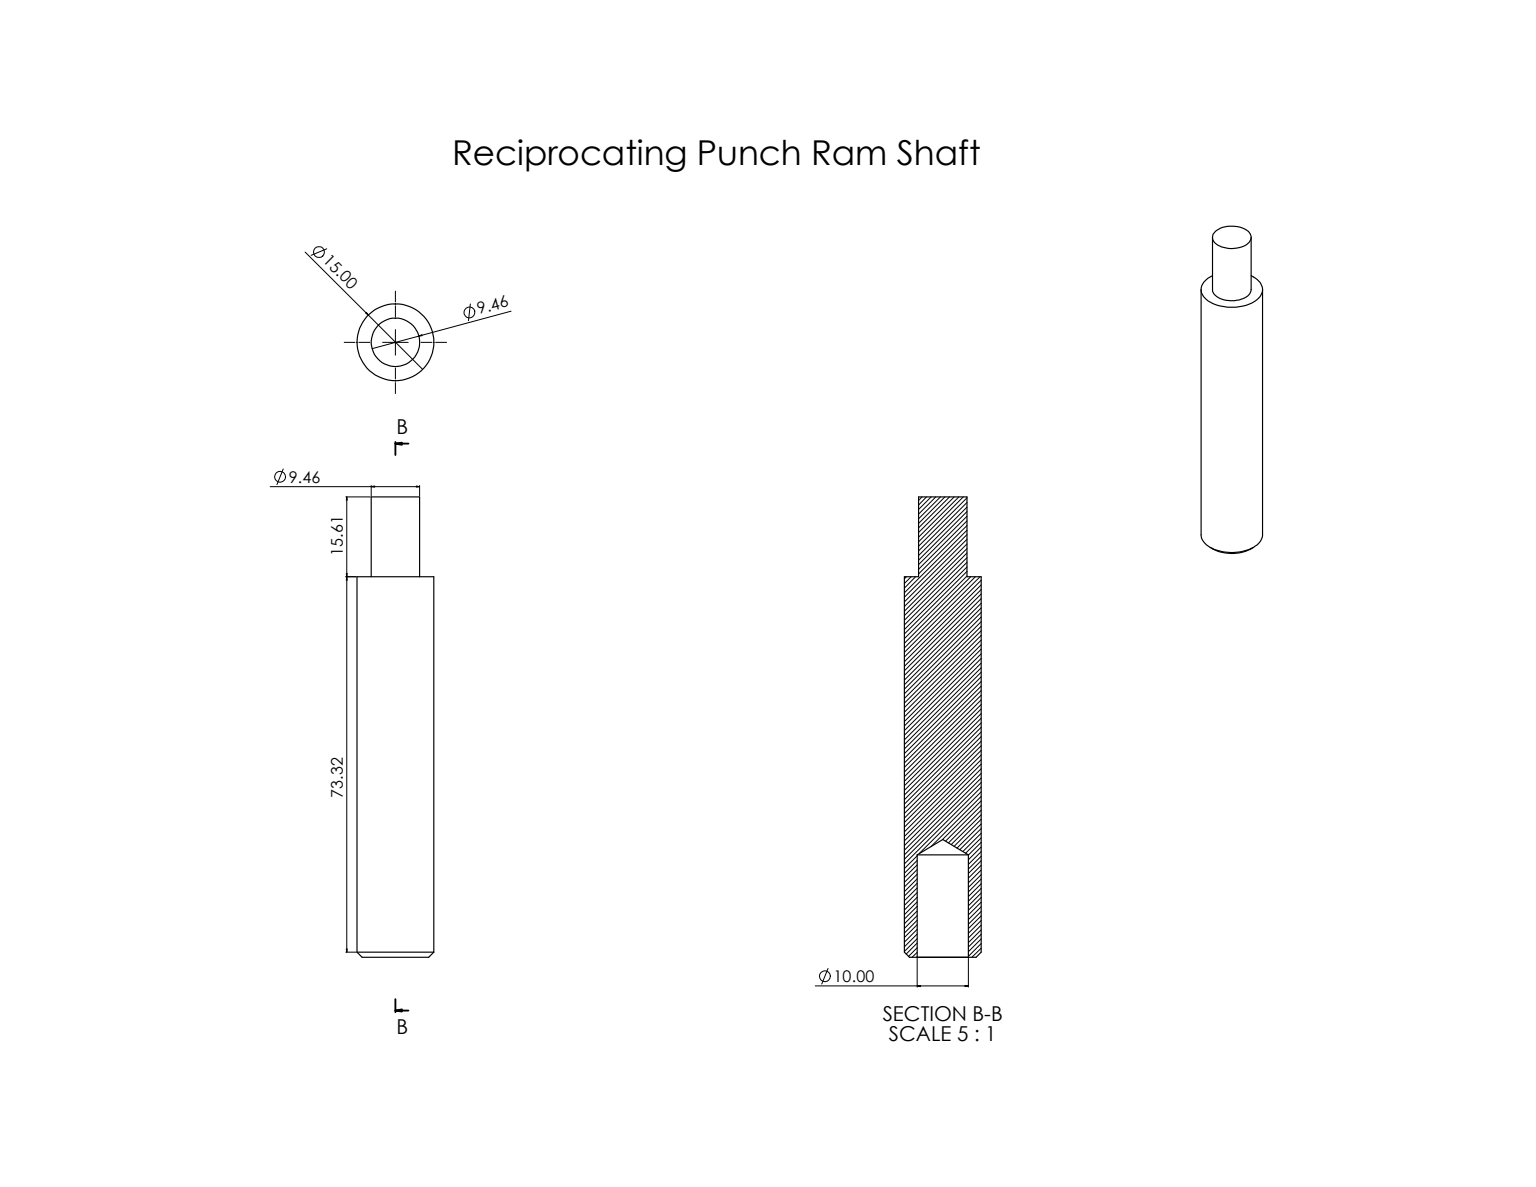
ISO-10303-21;
HEADER;
FILE_DESCRIPTION (('STEP AP214'),
    '1' );
FILE_NAME ('Reciprocating Punch Ram Shaft.step',
    '2026-10-20T14:49:59',
    ( '' ),
    ( '' ),
    'SwSTEP 2.0',
    'SolidWorks 2025',
    '' );
FILE_SCHEMA (( 'AUTOMOTIVE_DESIGN' ));
ENDSEC;

DATA;
#60=ORIENTED_EDGE ( 'NONE', *, *, #10146, .T. ) ;
#83=CIRCLE ( 'NONE', #590, 5.025000000000002132 ) ;
#136=CARTESIAN_POINT ( 'NONE',  ( -16.29350689640809691, -8.635287962196477096, 0.000000000000000000 ) ) ;
#199=DIRECTION ( 'NONE',  ( 0.000000000000000000, 0.000000000000000000, -1.000000000000000000 ) ) ;
#202=DIRECTION ( 'NONE',  ( 0.000000000000000000, 0.000000000000000000, -1.000000000000000000 ) ) ;
#307=CLOSED_SHELL ( 'NONE', ( #4177, #2796, #9152, #8006, #10397, #7112, #488, #9693, #5992, #7606, #7526, #5005, #9842, #7992, #7050 ) ) ;
#333=CARTESIAN_POINT ( 'NONE',  ( -16.29350689640809691, 81.26698356513965393, -4.729641367753003145 ) ) ;
#342=DIRECTION ( 'NONE',  ( 0.000000000000000000, 0.000000000000000000, -1.000000000000000000 ) ) ;
#358=DIRECTION ( 'NONE',  ( -0.000000000000000000, -1.000000000000000000, -0.000000000000000000 ) ) ;
#393=DIRECTION ( 'NONE',  ( -0.000000000000000000, -1.000000000000000000, -0.000000000000000000 ) ) ;
#447=FACE_OUTER_BOUND ( 'NONE', #1757, .T. ) ;
#471=( NAMED_UNIT ( * ) PLANE_ANGLE_UNIT ( ) SI_UNIT ( $, .RADIAN. ) );
#488=ADVANCED_FACE ( 'NONE', ( #4569, #3620 ), #8489, .T. ) ;
#509=FACE_OUTER_BOUND ( 'NONE', #4315, .T. ) ;
#517=EDGE_LOOP ( 'NONE', ( #2540, #3585, #6858, #7797 ) ) ;
#577=VECTOR ( 'NONE', #1492, 1000.000000000000000 ) ;
#590=AXIS2_PLACEMENT_3D ( 'NONE', #6539, #4054, #8179 ) ;
#625=DIRECTION ( 'NONE',  ( 0.000000000000000000, 0.000000000000000000, -1.000000000000000000 ) ) ;
#652=ORIENTED_EDGE ( 'NONE', *, *, #2869, .T. ) ;
#715=DIRECTION ( 'NONE',  ( 0.000000000000000000, 0.000000000000000000, -1.000000000000000000 ) ) ;
#719=VERTEX_POINT ( 'NONE', #3233 ) ;
#739=DIRECTION ( 'NONE',  ( 0.000000000000000000, 1.000000000000000000, 0.000000000000000000 ) ) ;
#755=CARTESIAN_POINT ( 'NONE',  ( -16.29350689640810401, 14.34401513294132613, 0.000000000000000000 ) ) ;
#789=EDGE_CURVE ( 'NONE', #10120, #2699, #7933, .T. ) ;
#851=DIRECTION ( 'NONE',  ( -0.000000000000000000, -1.000000000000000000, -0.000000000000000000 ) ) ;
#886=ORIENTED_EDGE ( 'NONE', *, *, #4179, .T. ) ;
#912=CIRCLE ( 'NONE', #6843, 7.499999999999998224 ) ;
#925=ORIENTED_EDGE ( 'NONE', *, *, #3802, .T. ) ;
#970=AXIS2_PLACEMENT_3D ( 'NONE', #4406, #7635, #2757 ) ;
#973=DIRECTION ( 'NONE',  ( 0.000000000000000000, 0.000000000000000000, -1.000000000000000000 ) ) ;
#989=FACE_OUTER_BOUND ( 'NONE', #8861, .T. ) ;
#1063=ORIENTED_EDGE ( 'NONE', *, *, #10418, .T. ) ;
#1067=CONICAL_SURFACE ( 'NONE', #8344, 4.999999999999993783, 1.029744258676652979 ) ;
#1068=EDGE_CURVE ( 'NONE', #2989, #5742, #4960, .T. ) ;
#1091=CARTESIAN_POINT ( 'NONE',  ( -16.29350689640809691, -8.635287962196477096, 0.000000000000000000 ) ) ;
#1125=DIRECTION ( 'NONE',  ( 0.000000000000000000, 0.000000000000000000, -1.000000000000000000 ) ) ;
#1128=EDGE_CURVE ( 'NONE', #5742, #6927, #4806, .T. ) ;
#1170=CONICAL_SURFACE ( 'NONE', #10140, 5.025000000000002132, 0.7853981633975176679 ) ;
#1207=CARTESIAN_POINT ( 'NONE',  ( -16.29350689640809691, -8.660287962196477451, 0.000000000000000000 ) ) ;
#1235=CARTESIAN_POINT ( 'NONE',  ( -16.29350689640809691, -8.660287962196477451, 7.499999999999998224 ) ) ;
#1236=CARTESIAN_POINT ( 'NONE',  ( -16.29350689640809691, 11.33971203780352255, 4.999999999999993783 ) ) ;
#1371=CARTESIAN_POINT ( 'NONE',  ( -16.29350689640809691, 81.26698356513965393, 0.000000000000000000 ) ) ;
#1378=( NAMED_UNIT ( * ) SI_UNIT ( $, .STERADIAN. ) SOLID_ANGLE_UNIT ( ) );
#1399=CONICAL_SURFACE ( 'NONE', #5616, 6.499999999999964473, 0.7853981633974560506 ) ;
#1426=CARTESIAN_POINT ( 'NONE',  ( -16.29350689640809691, 11.33971203780352255, -4.999999999999993783 ) ) ;
#1443=VERTEX_POINT ( 'NONE', #6181 ) ;
#1492=DIRECTION ( 'NONE',  ( 0.000000000000000000, -0.7071067811864985009, -0.7071067811865965336 ) ) ;
#1503=FACE_OUTER_BOUND ( 'NONE', #5938, .T. ) ;
#1513=CARTESIAN_POINT ( 'NONE',  ( -16.29350689640809691, 81.26698356513965393, 0.000000000000000000 ) ) ;
#1523=( GEOMETRIC_REPRESENTATION_CONTEXT ( 3 ) GLOBAL_UNCERTAINTY_ASSIGNED_CONTEXT ( ( #4366 ) ) GLOBAL_UNIT_ASSIGNED_CONTEXT ( ( #8417, #471, #3489 ) ) REPRESENTATION_CONTEXT ( 'NONE', 'WORKASPACE' ) );
#1665=CARTESIAN_POINT ( 'NONE',  ( -16.29350689640809691, -8.660287962196477451, 5.025000000000002132 ) ) ;
#1711=EDGE_CURVE ( 'NONE', #5823, #5289, #7017, .T. ) ;
#1733=AXIS2_PLACEMENT_3D ( 'NONE', #7041, #8623, #6238 ) ;
#1757=EDGE_LOOP ( 'NONE', ( #4011, #652, #8539, #8069 ) ) ;
#1781=CARTESIAN_POINT ( 'NONE',  ( -16.29350689640809691, -7.660287962196459688, 0.000000000000000000 ) ) ;
#1785=PRODUCT_DEFINITION ( 'UNKNOWN', '', #7350, #6637 ) ;
#1789=AXIS2_PLACEMENT_3D ( 'NONE', #9467, #7818, #715 ) ;
#1925=ORIENTED_EDGE ( 'NONE', *, *, #7233, .F. ) ;
#1935=CARTESIAN_POINT ( 'NONE',  ( -16.29350689640809691, -8.660287962196477451, -5.025000000000002132 ) ) ;
#1953=ORIENTED_EDGE ( 'NONE', *, *, #1068, .F. ) ;
#1972=CARTESIAN_POINT ( 'NONE',  ( -16.29350689640809691, -8.660287962196477451, -4.729641367753004033 ) ) ;
#1978=CARTESIAN_POINT ( 'NONE',  ( -16.29350689640809691, -7.660287962196459688, 7.499999999999998224 ) ) ;
#1985=EDGE_LOOP ( 'NONE', ( #9762, #3927 ) ) ;
#2018=ADVANCED_BREP_SHAPE_REPRESENTATION ( '', ( #3318, #4601 ), #9900 ) ;
#2057=AXIS2_PLACEMENT_3D ( 'NONE', #8439, #3780, #342 ) ;
#2064=VECTOR ( 'NONE', #8535, 1000.000000000000000 ) ;
#2078=DIRECTION ( 'NONE',  ( -0.000000000000000000, -1.000000000000000000, -0.000000000000000000 ) ) ;
#2079=AXIS2_PLACEMENT_3D ( 'NONE', #2227, #7159, #8636 ) ;
#2130=CARTESIAN_POINT ( 'NONE',  ( -16.29350689640809691, -8.660287962196477451, -6.499999999999964473 ) ) ;
#2190=LINE ( 'NONE', #6797, #8845 ) ;
#2227=CARTESIAN_POINT ( 'NONE',  ( -16.29350689640809691, -8.660287962196477451, 0.000000000000000000 ) ) ;
#2332=ORIENTED_EDGE ( 'NONE', *, *, #7411, .T. ) ;
#2367=DIRECTION ( 'NONE',  ( -0.000000000000000000, -1.000000000000000000, -0.000000000000000000 ) ) ;
#2378=LINE ( 'NONE', #8800, #577 ) ;
#2449=EDGE_CURVE ( 'NONE', #9987, #8969, #3678, .T. ) ;
#2530=ORIENTED_EDGE ( 'NONE', *, *, #5258, .T. ) ;
#2540=ORIENTED_EDGE ( 'NONE', *, *, #6007, .F. ) ;
#2575=AXIS2_PLACEMENT_3D ( 'NONE', #8320, #4873, #7320 ) ;
#2597=ORIENTED_EDGE ( 'NONE', *, *, #8641, .F. ) ;
#2599=CARTESIAN_POINT ( 'NONE',  ( -16.29350689640809691, -8.660287962196477451, 0.000000000000000000 ) ) ;
#2689=CIRCLE ( 'NONE', #8275, 7.499999999999996447 ) ;
#2699=VERTEX_POINT ( 'NONE', #3312 ) ;
#2706=ORIENTED_EDGE ( 'NONE', *, *, #8541, .T. ) ;
#2757=DIRECTION ( 'NONE',  ( 0.000000000000000000, 0.000000000000000000, -1.000000000000000000 ) ) ;
#2781=DIRECTION ( 'NONE',  ( -0.000000000000000000, -1.000000000000000000, -0.000000000000000000 ) ) ;
#2796=ADVANCED_FACE ( 'NONE', ( #6803 ), #1170, .F. ) ;
#2806=DIRECTION ( 'NONE',  ( 0.000000000000000000, 0.000000000000000000, -1.000000000000000000 ) ) ;
#2836=DIRECTION ( 'NONE',  ( 0.000000000000000000, 0.000000000000000000, -1.000000000000000000 ) ) ;
#2869=EDGE_CURVE ( 'NONE', #5823, #719, #2689, .T. ) ;
#2875=CARTESIAN_POINT ( 'NONE',  ( -16.29350689640809691, -8.660287962196477451, 0.000000000000000000 ) ) ;
#2884=DIRECTION ( 'NONE',  ( 0.000000000000000000, 0.000000000000000000, -1.000000000000000000 ) ) ;
#2896=CIRCLE ( 'NONE', #5605, 4.999999999999997335 ) ;
#2940=CIRCLE ( 'NONE', #9381, 4.999999999999993783 ) ;
#2956=ORIENTED_EDGE ( 'NONE', *, *, #7233, .T. ) ;
#2989=VERTEX_POINT ( 'NONE', #755 ) ;
#2990=ORIENTED_EDGE ( 'NONE', *, *, #1128, .F. ) ;
#3002=ORIENTED_EDGE ( 'NONE', *, *, #8980, .T. ) ;
#3003=DIRECTION ( 'NONE',  ( 0.000000000000000000, 0.000000000000000000, -1.000000000000000000 ) ) ;
#3065=ORIENTED_EDGE ( 'NONE', *, *, #1068, .T. ) ;
#3090=VECTOR ( 'NONE', #5324, 1000.000000000000000 ) ;
#3103=SHAPE_DEFINITION_REPRESENTATION ( #10435, #3996 ) ;
#3176=FACE_OUTER_BOUND ( 'NONE', #9339, .T. ) ;
#3233=CARTESIAN_POINT ( 'NONE',  ( -16.29350689640809691, 65.65569765742554864, -7.499999999999996447 ) ) ;
#3268=CIRCLE ( 'NONE', #3951, 4.999999999999993783 ) ;
#3299=ORIENTED_EDGE ( 'NONE', *, *, #8980, .F. ) ;
#3312=CARTESIAN_POINT ( 'NONE',  ( -16.29350689640809691, -8.660287962196477451, 6.499999999999964473 ) ) ;
#3318=MANIFOLD_SOLID_BREP ( 'Chamfer1', #307 ) ;
#3365=AXIS2_PLACEMENT_3D ( 'NONE', #2599, #5982, #3715 ) ;
#3433=EDGE_LOOP ( 'NONE', ( #3804, #1063, #3002, #4595 ) ) ;
#3489=( NAMED_UNIT ( * ) SI_UNIT ( $, .STERADIAN. ) SOLID_ANGLE_UNIT ( ) );
#3584=CARTESIAN_POINT ( 'NONE',  ( -16.29350689640809691, -8.660287962196477451, 4.999999999999995559 ) ) ;
#3585=ORIENTED_EDGE ( 'NONE', *, *, #7838, .F. ) ;
#3620=FACE_BOUND ( 'NONE', #9058, .T. ) ;
#3674=ORIENTED_EDGE ( 'NONE', *, *, #7437, .T. ) ;
#3678=CIRCLE ( 'NONE', #9612, 4.729641367753004921 ) ;
#3715=DIRECTION ( 'NONE',  ( 0.000000000000000000, 0.000000000000000000, -1.000000000000000000 ) ) ;
#3723=ORIENTED_EDGE ( 'NONE', *, *, #4733, .F. ) ;
#3730=LINE ( 'NONE', #1972, #5285 ) ;
#3745=ORIENTED_EDGE ( 'NONE', *, *, #4405, .F. ) ;
#3767=CIRCLE ( 'NONE', #9695, 4.999999999999997335 ) ;
#3780=DIRECTION ( 'NONE',  ( -0.000000000000000000, -1.000000000000000000, -0.000000000000000000 ) ) ;
#3802=EDGE_CURVE ( 'NONE', #4078, #1443, #4189, .T. ) ;
#3804=ORIENTED_EDGE ( 'NONE', *, *, #7322, .F. ) ;
#3927=ORIENTED_EDGE ( 'NONE', *, *, #7379, .F. ) ;
#3948=ORIENTED_EDGE ( 'NONE', *, *, #4048, .T. ) ;
#3951=AXIS2_PLACEMENT_3D ( 'NONE', #6581, #9824, #9015 ) ;
#3980=EDGE_CURVE ( 'NONE', #8969, #9987, #6222, .T. ) ;
#3996=SHAPE_REPRESENTATION ( 'Reciprocating Punch Ram Shaft', ( #4601 ), #9900 ) ;
#4011=ORIENTED_EDGE ( 'NONE', *, *, #1711, .F. ) ;
#4048=EDGE_CURVE ( 'NONE', #5289, #9924, #5370, .T. ) ;
#4054=DIRECTION ( 'NONE',  ( -0.000000000000000000, -1.000000000000000000, -0.000000000000000000 ) ) ;
#4078=VERTEX_POINT ( 'NONE', #333 ) ;
#4119=CYLINDRICAL_SURFACE ( 'NONE', #8143, 4.999999999999995559 ) ;
#4177=ADVANCED_FACE ( 'NONE', ( #10296 ), #7531, .T. ) ;
#4178=CARTESIAN_POINT ( 'NONE',  ( -16.29350689640809691, -8.635287962196477096, -4.999999999999997335 ) ) ;
#4179=EDGE_CURVE ( 'NONE', #6927, #8802, #2378, .T. ) ;
#4189=CIRCLE ( 'NONE', #7404, 4.729641367753003145 ) ;
#4206=CARTESIAN_POINT ( 'NONE',  ( -16.29350689640809691, 65.65569765742554864, 4.729641367753004921 ) ) ;
#4212=ORIENTED_EDGE ( 'NONE', *, *, #4733, .T. ) ;
#4234=DIRECTION ( 'NONE',  ( -0.000000000000000000, -1.000000000000000000, -0.000000000000000000 ) ) ;
#4267=CIRCLE ( 'NONE', #1733, 7.499999999999996447 ) ;
#4272=LINE ( 'NONE', #8194, #8046 ) ;
#4315=EDGE_LOOP ( 'NONE', ( #9603, #3065, #9285 ) ) ;
#4366=UNCERTAINTY_MEASURE_WITH_UNIT (LENGTH_MEASURE( 1.000000000000000082E-05 ), #8417, 'distance_accuracy_value', 'NONE');
#4368=DIRECTION ( 'NONE',  ( 0.000000000000000000, 0.7071067811865420216, 0.7071067811865531239 ) ) ;
#4405=EDGE_CURVE ( 'NONE', #719, #9924, #5818, .T. ) ;
#4406=CARTESIAN_POINT ( 'NONE',  ( -16.29350689640809691, -7.660287962196459688, 0.000000000000000000 ) ) ;
#4412=DIRECTION ( 'NONE',  ( -0.000000000000000000, -1.000000000000000000, -0.000000000000000000 ) ) ;
#4413=DIRECTION ( 'NONE',  ( -0.000000000000000000, -1.000000000000000000, -0.000000000000000000 ) ) ;
#4418=AXIS2_PLACEMENT_3D ( 'NONE', #1371, #8788, #10433 ) ;
#4439=DIRECTION ( 'NONE',  ( 0.000000000000000000, 1.000000000000000000, 0.000000000000000000 ) ) ;
#4446=AXIS2_PLACEMENT_3D ( 'NONE', #4594, #7096, #625 ) ;
#4459=ORIENTED_EDGE ( 'NONE', *, *, #789, .T. ) ;
#4487=CARTESIAN_POINT ( 'NONE',  ( -16.29350689640809691, 65.65569765742554864, 0.000000000000000000 ) ) ;
#4528=DIRECTION ( 'NONE',  ( -0.000000000000000000, -1.000000000000000000, -0.000000000000000000 ) ) ;
#4555=ORIENTED_EDGE ( 'NONE', *, *, #789, .F. ) ;
#4569=FACE_OUTER_BOUND ( 'NONE', #7092, .T. ) ;
#4577=CARTESIAN_POINT ( 'NONE',  ( -16.29350689640809691, 65.65569765742554864, 0.000000000000000000 ) ) ;
#4586=PRODUCT_CONTEXT ( 'NONE', #8219, 'mechanical' ) ;
#4594=CARTESIAN_POINT ( 'NONE',  ( -16.29350689640809691, -8.660287962196477451, 0.000000000000000000 ) ) ;
#4595=ORIENTED_EDGE ( 'NONE', *, *, #4179, .F. ) ;
#4601=AXIS2_PLACEMENT_3D ( 'NONE', #8586, #5983, #5928 ) ;
#4651=DIRECTION ( 'NONE',  ( 0.000000000000000000, 0.000000000000000000, -1.000000000000000000 ) ) ;
#4733=EDGE_CURVE ( 'NONE', #10120, #9924, #4272, .T. ) ;
#4802=ORIENTED_EDGE ( 'NONE', *, *, #3980, .F. ) ;
#4806=LINE ( 'NONE', #5756, #9115 ) ;
#4823=DIRECTION ( 'NONE',  ( 0.000000000000000000, -0.000000000000000000, 1.000000000000000000 ) ) ;
#4873=DIRECTION ( 'NONE',  ( -0.000000000000000000, -1.000000000000000000, -0.000000000000000000 ) ) ;
#4874=FACE_BOUND ( 'NONE', #7735, .T. ) ;
#4945=AXIS2_PLACEMENT_3D ( 'NONE', #8058, #7173, #4823 ) ;
#4960=LINE ( 'NONE', #9701, #7251 ) ;
#4970=EDGE_LOOP ( 'NONE', ( #2956, #7579, #3948, #3745 ) ) ;
#4994=CONICAL_SURFACE ( 'NONE', #1789, 4.999999999999993783, 1.029744258676652979 ) ;
#5005=ADVANCED_FACE ( 'NONE', ( #509 ), #4994, .F. ) ;
#5027=EDGE_LOOP ( 'NONE', ( #6272, #5643, #6069, #2990 ) ) ;
#5047=DIRECTION ( 'NONE',  ( -0.000000000000000000, -1.000000000000000000, -0.000000000000000000 ) ) ;
#5065=MECHANICAL_DESIGN_GEOMETRIC_PRESENTATION_REPRESENTATION('',(#6941),#1523);
#5078=ORIENTED_EDGE ( 'NONE', *, *, #7379, .T. ) ;
#5087=FACE_OUTER_BOUND ( 'NONE', #4970, .T. ) ;
#5121=CIRCLE ( 'NONE', #8338, 4.729641367753003145 ) ;
#5195=ORIENTED_EDGE ( 'NONE', *, *, #9887, .F. ) ;
#5215=DIRECTION ( 'NONE',  ( 0.000000000000000000, 0.000000000000000000, -1.000000000000000000 ) ) ;
#5256=ORIENTED_EDGE ( 'NONE', *, *, #7437, .F. ) ;
#5258=EDGE_CURVE ( 'NONE', #2699, #5289, #6798, .T. ) ;
#5267=FACE_OUTER_BOUND ( 'NONE', #517, .T. ) ;
#5285=VECTOR ( 'NONE', #4413, 1000.000000000000000 ) ;
#5289=VERTEX_POINT ( 'NONE', #1978 ) ;
#5308=DIRECTION ( 'NONE',  ( 0.000000000000000000, 0.000000000000000000, -1.000000000000000000 ) ) ;
#5324=DIRECTION ( 'NONE',  ( -0.000000000000000000, -1.000000000000000000, -0.000000000000000000 ) ) ;
#5330=EDGE_LOOP ( 'NONE', ( #6438, #5195, #886, #9735 ) ) ;
#5369=CARTESIAN_POINT ( 'NONE',  ( -16.29350689640809691, -8.660287962196477451, 0.000000000000000000 ) ) ;
#5370=CIRCLE ( 'NONE', #970, 7.499999999999998224 ) ;
#5605=AXIS2_PLACEMENT_3D ( 'NONE', #1091, #2781, #2836 ) ;
#5608=LINE ( 'NONE', #7901, #5806 ) ;
#5616=AXIS2_PLACEMENT_3D ( 'NONE', #1207, #4439, #8520 ) ;
#5643=ORIENTED_EDGE ( 'NONE', *, *, #6007, .T. ) ;
#5731=ORIENTED_EDGE ( 'NONE', *, *, #10146, .F. ) ;
#5742=VERTEX_POINT ( 'NONE', #1426 ) ;
#5756=CARTESIAN_POINT ( 'NONE',  ( -16.29350689640809691, -8.660287962196477451, -4.999999999999995559 ) ) ;
#5806=VECTOR ( 'NONE', #6406, 1000.000000000000000 ) ;
#5818=LINE ( 'NONE', #9055, #9398 ) ;
#5823=VERTEX_POINT ( 'NONE', #6845 ) ;
#5908=CARTESIAN_POINT ( 'NONE',  ( -16.29350689640809691, -7.660287962196459688, -7.499999999999998224 ) ) ;
#5928=DIRECTION ( 'NONE',  ( 1.000000000000000000, 0.000000000000000000, 0.000000000000000000 ) ) ;
#5938=EDGE_LOOP ( 'NONE', ( #1925, #6340 ) ) ;
#5940=DIRECTION ( 'NONE',  ( 0.000000000000000000, -1.000000000000000000, -0.000000000000000000 ) ) ;
#5959=DIRECTION ( 'NONE',  ( 0.000000000000000000, 0.000000000000000000, -1.000000000000000000 ) ) ;
#5982=DIRECTION ( 'NONE',  ( -0.000000000000000000, -1.000000000000000000, -0.000000000000000000 ) ) ;
#5983=DIRECTION ( 'NONE',  ( 0.000000000000000000, 0.000000000000000000, 1.000000000000000000 ) ) ;
#5992=ADVANCED_FACE ( 'NONE', ( #989 ), #6607, .T. ) ;
#6007=EDGE_CURVE ( 'NONE', #7514, #9202, #6712, .T. ) ;
#6044=AXIS2_PLACEMENT_3D ( 'NONE', #10240, #9387, #2806 ) ;
#6069=ORIENTED_EDGE ( 'NONE', *, *, #7322, .T. ) ;
#6103=DIRECTION ( 'NONE',  ( 0.000000000000000000, 0.000000000000000000, -1.000000000000000000 ) ) ;
#6174=ORIENTED_EDGE ( 'NONE', *, *, #5258, .F. ) ;
#6181=CARTESIAN_POINT ( 'NONE',  ( -16.29350689640809691, 81.26698356513965393, 4.729641367753003145 ) ) ;
#6222=CIRCLE ( 'NONE', #6044, 4.729641367753004921 ) ;
#6238=DIRECTION ( 'NONE',  ( 0.000000000000000000, 0.000000000000000000, -1.000000000000000000 ) ) ;
#6259=CARTESIAN_POINT ( 'NONE',  ( -16.29350689640809691, -8.635287962196477096, 4.999999999999998224 ) ) ;
#6272=ORIENTED_EDGE ( 'NONE', *, *, #8541, .F. ) ;
#6321=CONICAL_SURFACE ( 'NONE', #2079, 5.025000000000002132, 0.7853981633975176679 ) ;
#6340=ORIENTED_EDGE ( 'NONE', *, *, #2869, .F. ) ;
#6406=DIRECTION ( 'NONE',  ( -0.000000000000000000, -1.000000000000000000, -0.000000000000000000 ) ) ;
#6438=ORIENTED_EDGE ( 'NONE', *, *, #10418, .F. ) ;
#6532=UNCERTAINTY_MEASURE_WITH_UNIT (LENGTH_MEASURE( 1.000000000000000082E-05 ), #9441, 'distance_accuracy_value', 'NONE');
#6539=CARTESIAN_POINT ( 'NONE',  ( -16.29350689640809691, -8.660287962196477451, 0.000000000000000000 ) ) ;
#6577=ORIENTED_EDGE ( 'NONE', *, *, #9022, .F. ) ;
#6581=CARTESIAN_POINT ( 'NONE',  ( -16.29350689640809691, 11.33971203780352255, 0.000000000000000000 ) ) ;
#6607=CYLINDRICAL_SURFACE ( 'NONE', #7998, 4.729641367753004033 ) ;
#6608=ORIENTED_EDGE ( 'NONE', *, *, #8049, .F. ) ;
#6625=CIRCLE ( 'NONE', #2057, 6.499999999999964473 ) ;
#6637=PRODUCT_DEFINITION_CONTEXT ( 'detailed design', #7882, 'design' ) ;
#6712=LINE ( 'NONE', #3584, #3090 ) ;
#6781=CARTESIAN_POINT ( 'NONE',  ( -16.29350689640809691, -8.660287962196477451, 5.025000000000002132 ) ) ;
#6797=CARTESIAN_POINT ( 'NONE',  ( -16.29350689640809691, 11.33971203780352255, 4.999999999999993783 ) ) ;
#6798=LINE ( 'NONE', #10039, #9598 ) ;
#6803=FACE_OUTER_BOUND ( 'NONE', #3433, .T. ) ;
#6843=AXIS2_PLACEMENT_3D ( 'NONE', #1781, #8939, #199 ) ;
#6845=CARTESIAN_POINT ( 'NONE',  ( -16.29350689640809691, 65.65569765742554864, 7.499999999999996447 ) ) ;
#6858=ORIENTED_EDGE ( 'NONE', *, *, #1128, .T. ) ;
#6917=DIRECTION ( 'NONE',  ( -0.000000000000000000, -1.000000000000000000, -0.000000000000000000 ) ) ;
#6925=ORIENTED_EDGE ( 'NONE', *, *, #8049, .T. ) ;
#6927=VERTEX_POINT ( 'NONE', #4178 ) ;
#6941=STYLED_ITEM('',(#10518),#3318);
#6951=DIRECTION ( 'NONE',  ( 0.000000000000000000, 0.000000000000000000, -1.000000000000000000 ) ) ;
#7014=CARTESIAN_POINT ( 'NONE',  ( -8.793506896408096907, -8.660287962196477451, 0.000000000000000000 ) ) ;
#7017=LINE ( 'NONE', #1235, #10097 ) ;
#7041=CARTESIAN_POINT ( 'NONE',  ( -16.29350689640809691, 65.65569765742554864, 0.000000000000000000 ) ) ;
#7050=ADVANCED_FACE ( 'NONE', ( #8467 ), #1399, .T. ) ;
#7092=EDGE_LOOP ( 'NONE', ( #60, #4459 ) ) ;
#7096=DIRECTION ( 'NONE',  ( -0.000000000000000000, -1.000000000000000000, -0.000000000000000000 ) ) ;
#7112=ADVANCED_FACE ( 'NONE', ( #7281 ), #9424, .T. ) ;
#7150=FACE_OUTER_BOUND ( 'NONE', #1985, .T. ) ;
#7154=ORIENTED_EDGE ( 'NONE', *, *, #2449, .T. ) ;
#7159=DIRECTION ( 'NONE',  ( -0.000000000000000000, -1.000000000000000000, -0.000000000000000000 ) ) ;
#7171=VERTEX_POINT ( 'NONE', #1665 ) ;
#7173=DIRECTION ( 'NONE',  ( 0.000000000000000000, 1.000000000000000000, 0.000000000000000000 ) ) ;
#7209=DIRECTION ( 'NONE',  ( 0.000000000000000000, 0.000000000000000000, 1.000000000000000000 ) ) ;
#7233=EDGE_CURVE ( 'NONE', #719, #5823, #4267, .T. ) ;
#7251=VECTOR ( 'NONE', #9052, 1000.000000000000000 ) ;
#7261=FACE_OUTER_BOUND ( 'NONE', #5330, .T. ) ;
#7281=FACE_OUTER_BOUND ( 'NONE', #9671, .T. ) ;
#7298=CARTESIAN_POINT ( 'NONE',  ( -16.29350689640809691, -8.660287962196477451, 0.000000000000000000 ) ) ;
#7320=DIRECTION ( 'NONE',  ( 0.000000000000000000, 0.000000000000000000, -1.000000000000000000 ) ) ;
#7322=EDGE_CURVE ( 'NONE', #9202, #6927, #3767, .T. ) ;
#7328=ORIENTED_EDGE ( 'NONE', *, *, #2449, .F. ) ;
#7350=PRODUCT_DEFINITION_FORMATION_WITH_SPECIFIED_SOURCE ( 'ANY', '', #9406, .NOT_KNOWN. ) ;
#7379=EDGE_CURVE ( 'NONE', #1443, #4078, #5121, .T. ) ;
#7404=AXIS2_PLACEMENT_3D ( 'NONE', #1513, #851, #2884 ) ;
#7411=EDGE_CURVE ( 'NONE', #2989, #7514, #2190, .T. ) ;
#7437=EDGE_CURVE ( 'NONE', #4078, #8969, #3730, .T. ) ;
#7453=ORIENTED_EDGE ( 'NONE', *, *, #4048, .F. ) ;
#7458=DIRECTION ( 'NONE',  ( -0.000000000000000000, -1.000000000000000000, -0.000000000000000000 ) ) ;
#7514=VERTEX_POINT ( 'NONE', #1236 ) ;
#7526=ADVANCED_FACE ( 'NONE', ( #447 ), #10144, .T. ) ;
#7531=CONICAL_SURFACE ( 'NONE', #9742, 6.499999999999964473, 0.7853981633974560506 ) ;
#7544=DIRECTION ( 'NONE',  ( 0.000000000000000000, 0.000000000000000000, -1.000000000000000000 ) ) ;
#7579=ORIENTED_EDGE ( 'NONE', *, *, #1711, .T. ) ;
#7606=ADVANCED_FACE ( 'NONE', ( #4874, #1503 ), #7964, .T. ) ;
#7635=DIRECTION ( 'NONE',  ( 0.000000000000000000, 1.000000000000000000, 0.000000000000000000 ) ) ;
#7681=EDGE_LOOP ( 'NONE', ( #3723, #5731, #2530, #2597 ) ) ;
#7695=AXIS2_PLACEMENT_3D ( 'NONE', #9030, #9678, #973 ) ;
#7735=EDGE_LOOP ( 'NONE', ( #7772, #7154 ) ) ;
#7757=DIRECTION ( 'NONE',  ( 1.049727191138617710E-16, -0.5150380749100554878, 0.8571673007021115565 ) ) ;
#7772=ORIENTED_EDGE ( 'NONE', *, *, #3980, .T. ) ;
#7797=ORIENTED_EDGE ( 'NONE', *, *, #9887, .T. ) ;
#7818=DIRECTION ( 'NONE',  ( -0.000000000000000000, -1.000000000000000000, -0.000000000000000000 ) ) ;
#7838=EDGE_CURVE ( 'NONE', #5742, #7514, #3268, .T. ) ;
#7847=CYLINDRICAL_SURFACE ( 'NONE', #8368, 4.999999999999995559 ) ;
#7882=APPLICATION_CONTEXT ( 'automotive_design' ) ;
#7901=CARTESIAN_POINT ( 'NONE',  ( -16.29350689640809691, -8.660287962196477451, 4.729641367753004033 ) ) ;
#7933=CIRCLE ( 'NONE', #3365, 6.499999999999964473 ) ;
#7954=CARTESIAN_POINT ( 'NONE',  ( -16.29350689640809691, 11.33971203780352255, 0.000000000000000000 ) ) ;
#7964=PLANE ( 'NONE',  #4945 ) ;
#7992=ADVANCED_FACE ( 'NONE', ( #7261 ), #6321, .F. ) ;
#7998=AXIS2_PLACEMENT_3D ( 'NONE', #7298, #7458, #202 ) ;
#8006=ADVANCED_FACE ( 'NONE', ( #3176 ), #1067, .F. ) ;
#8046=VECTOR ( 'NONE', #9045, 999.9999999999998863 ) ;
#8049=EDGE_CURVE ( 'NONE', #1443, #9987, #5608, .T. ) ;
#8058=CARTESIAN_POINT ( 'NONE',  ( -11.56386552865509110, 65.65569765742554864, 0.000000000000000000 ) ) ;
#8069=ORIENTED_EDGE ( 'NONE', *, *, #8641, .T. ) ;
#8143=AXIS2_PLACEMENT_3D ( 'NONE', #9254, #358, #5959 ) ;
#8179=DIRECTION ( 'NONE',  ( 0.000000000000000000, 0.000000000000000000, -1.000000000000000000 ) ) ;
#8194=CARTESIAN_POINT ( 'NONE',  ( -16.29350689640809691, -8.660287962196477451, -6.499999999999964473 ) ) ;
#8219=APPLICATION_CONTEXT ( 'automotive_design' ) ;
#8275=AXIS2_PLACEMENT_3D ( 'NONE', #4577, #6917, #5215 ) ;
#8320=CARTESIAN_POINT ( 'NONE',  ( -16.29350689640809691, -8.660287962196477451, 0.000000000000000000 ) ) ;
#8338=AXIS2_PLACEMENT_3D ( 'NONE', #8602, #393, #6103 ) ;
#8344=AXIS2_PLACEMENT_3D ( 'NONE', #7954, #8746, #10295 ) ;
#8368=AXIS2_PLACEMENT_3D ( 'NONE', #8392, #9446, #6951 ) ;
#8392=CARTESIAN_POINT ( 'NONE',  ( -16.29350689640809691, -8.660287962196477451, 0.000000000000000000 ) ) ;
#8417=( LENGTH_UNIT ( ) NAMED_UNIT ( * ) SI_UNIT ( .MILLI., .METRE. ) );
#8428=AXIS2_PLACEMENT_3D ( 'NONE', #7014, #5940, #1125 ) ;
#8439=CARTESIAN_POINT ( 'NONE',  ( -16.29350689640809691, -8.660287962196477451, 0.000000000000000000 ) ) ;
#8450=DIRECTION ( 'NONE',  ( 0.000000000000000000, 0.000000000000000000, -1.000000000000000000 ) ) ;
#8467=FACE_OUTER_BOUND ( 'NONE', #7681, .T. ) ;
#8477=LINE ( 'NONE', #6781, #2064 ) ;
#8489=PLANE ( 'NONE',  #8428 ) ;
#8520=DIRECTION ( 'NONE',  ( 0.000000000000000000, 0.000000000000000000, 1.000000000000000000 ) ) ;
#8535=DIRECTION ( 'NONE',  ( 8.659560562355533132E-17, -0.7071067811864985009, 0.7071067811865965336 ) ) ;
#8539=ORIENTED_EDGE ( 'NONE', *, *, #4405, .T. ) ;
#8541=EDGE_CURVE ( 'NONE', #7514, #5742, #2940, .T. ) ;
#8586=CARTESIAN_POINT ( 'NONE',  ( 0.000000000000000000, 0.000000000000000000, 0.000000000000000000 ) ) ;
#8602=CARTESIAN_POINT ( 'NONE',  ( -16.29350689640809691, 81.26698356513965393, 0.000000000000000000 ) ) ;
#8623=DIRECTION ( 'NONE',  ( -0.000000000000000000, -1.000000000000000000, -0.000000000000000000 ) ) ;
#8636=DIRECTION ( 'NONE',  ( 0.000000000000000000, 0.000000000000000000, -1.000000000000000000 ) ) ;
#8641=EDGE_CURVE ( 'NONE', #9924, #5289, #912, .T. ) ;
#8709=CIRCLE ( 'NONE', #7695, 5.025000000000002132 ) ;
#8746=DIRECTION ( 'NONE',  ( -0.000000000000000000, -1.000000000000000000, -0.000000000000000000 ) ) ;
#8747=CARTESIAN_POINT ( 'NONE',  ( -16.29350689640809691, -8.660287962196477451, 0.000000000000000000 ) ) ;
#8788=DIRECTION ( 'NONE',  ( 0.000000000000000000, 1.000000000000000000, 0.000000000000000000 ) ) ;
#8800=CARTESIAN_POINT ( 'NONE',  ( -16.29350689640809691, -8.660287962196477451, -5.025000000000002132 ) ) ;
#8802=VERTEX_POINT ( 'NONE', #1935 ) ;
#8817=CARTESIAN_POINT ( 'NONE',  ( -16.29350689640809691, 65.65569765742554864, -4.729641367753004921 ) ) ;
#8845=VECTOR ( 'NONE', #7757, 1000.000000000000000 ) ;
#8861=EDGE_LOOP ( 'NONE', ( #6608, #5078, #3674, #7328 ) ) ;
#8911=CYLINDRICAL_SURFACE ( 'NONE', #2575, 7.499999999999998224 ) ;
#8939=DIRECTION ( 'NONE',  ( 0.000000000000000000, 1.000000000000000000, 0.000000000000000000 ) ) ;
#8969=VERTEX_POINT ( 'NONE', #8817 ) ;
#8971=EDGE_LOOP ( 'NONE', ( #4555, #4212, #7453, #6174 ) ) ;
#8980=EDGE_CURVE ( 'NONE', #7171, #8802, #8709, .T. ) ;
#8999=DIRECTION ( 'NONE',  ( -0.000000000000000000, -1.000000000000000000, -0.000000000000000000 ) ) ;
#9015=DIRECTION ( 'NONE',  ( 0.000000000000000000, 0.000000000000000000, -1.000000000000000000 ) ) ;
#9022=EDGE_CURVE ( 'NONE', #8802, #7171, #83, .T. ) ;
#9030=CARTESIAN_POINT ( 'NONE',  ( -16.29350689640809691, -8.660287962196477451, 0.000000000000000000 ) ) ;
#9045=DIRECTION ( 'NONE',  ( 8.659560562355001884E-17, 0.7071067811865420216, -0.7071067811865531239 ) ) ;
#9052=DIRECTION ( 'NONE',  ( 0.000000000000000000, -0.5150380749100554878, -0.8571673007021115565 ) ) ;
#9055=CARTESIAN_POINT ( 'NONE',  ( -16.29350689640809691, -8.660287962196477451, -7.499999999999998224 ) ) ;
#9058=EDGE_LOOP ( 'NONE', ( #6577, #3299 ) ) ;
#9115=VECTOR ( 'NONE', #8999, 1000.000000000000000 ) ;
#9152=ADVANCED_FACE ( 'NONE', ( #9946 ), #7847, .F. ) ;
#9202=VERTEX_POINT ( 'NONE', #6259 ) ;
#9254=CARTESIAN_POINT ( 'NONE',  ( -16.29350689640809691, -8.660287962196477451, 0.000000000000000000 ) ) ;
#9285=ORIENTED_EDGE ( 'NONE', *, *, #7838, .T. ) ;
#9339=EDGE_LOOP ( 'NONE', ( #1953, #2332, #2706 ) ) ;
#9381=AXIS2_PLACEMENT_3D ( 'NONE', #10430, #2367, #4651 ) ;
#9387=DIRECTION ( 'NONE',  ( -0.000000000000000000, -1.000000000000000000, -0.000000000000000000 ) ) ;
#9398=VECTOR ( 'NONE', #4234, 1000.000000000000000 ) ;
#9406=PRODUCT ( 'Reciprocating Punch Ram Shaft', 'Reciprocating Punch Ram Shaft', '', ( #4586 ) ) ;
#9424=CYLINDRICAL_SURFACE ( 'NONE', #4446, 4.729641367753004033 ) ;
#9441=( LENGTH_UNIT ( ) NAMED_UNIT ( * ) SI_UNIT ( .MILLI., .METRE. ) );
#9446=DIRECTION ( 'NONE',  ( -0.000000000000000000, -1.000000000000000000, -0.000000000000000000 ) ) ;
#9467=CARTESIAN_POINT ( 'NONE',  ( -16.29350689640809691, 11.33971203780352255, 0.000000000000000000 ) ) ;
#9551=( NAMED_UNIT ( * ) PLANE_ANGLE_UNIT ( ) SI_UNIT ( $, .RADIAN. ) );
#9598=VECTOR ( 'NONE', #4368, 999.9999999999998863 ) ;
#9603=ORIENTED_EDGE ( 'NONE', *, *, #7411, .F. ) ;
#9612=AXIS2_PLACEMENT_3D ( 'NONE', #4487, #10271, #3003 ) ;
#9671=EDGE_LOOP ( 'NONE', ( #925, #6925, #4802, #5256 ) ) ;
#9678=DIRECTION ( 'NONE',  ( -0.000000000000000000, -1.000000000000000000, -0.000000000000000000 ) ) ;
#9693=ADVANCED_FACE ( 'NONE', ( #7150 ), #10383, .T. ) ;
#9695=AXIS2_PLACEMENT_3D ( 'NONE', #136, #5047, #7544 ) ;
#9701=CARTESIAN_POINT ( 'NONE',  ( -16.29350689640809691, 11.33971203780352255, -4.999999999999993783 ) ) ;
#9735=ORIENTED_EDGE ( 'NONE', *, *, #9022, .T. ) ;
#9742=AXIS2_PLACEMENT_3D ( 'NONE', #8747, #739, #7209 ) ;
#9762=ORIENTED_EDGE ( 'NONE', *, *, #3802, .F. ) ;
#9824=DIRECTION ( 'NONE',  ( -0.000000000000000000, -1.000000000000000000, -0.000000000000000000 ) ) ;
#9842=ADVANCED_FACE ( 'NONE', ( #5267 ), #4119, .F. ) ;
#9887=EDGE_CURVE ( 'NONE', #6927, #9202, #2896, .T. ) ;
#9900=( GEOMETRIC_REPRESENTATION_CONTEXT ( 3 ) GLOBAL_UNCERTAINTY_ASSIGNED_CONTEXT ( ( #6532 ) ) GLOBAL_UNIT_ASSIGNED_CONTEXT ( ( #9441, #9551, #1378 ) ) REPRESENTATION_CONTEXT ( 'NONE', 'WORKASPACE' ) );
#9924=VERTEX_POINT ( 'NONE', #5908 ) ;
#9946=FACE_OUTER_BOUND ( 'NONE', #5027, .T. ) ;
#9987=VERTEX_POINT ( 'NONE', #4206 ) ;
#10039=CARTESIAN_POINT ( 'NONE',  ( -16.29350689640809691, -8.660287962196477451, 6.499999999999964473 ) ) ;
#10097=VECTOR ( 'NONE', #4412, 1000.000000000000000 ) ;
#10120=VERTEX_POINT ( 'NONE', #2130 ) ;
#10140=AXIS2_PLACEMENT_3D ( 'NONE', #5369, #4528, #8450 ) ;
#10144=CYLINDRICAL_SURFACE ( 'NONE', #10382, 7.499999999999998224 ) ;
#10146=EDGE_CURVE ( 'NONE', #2699, #10120, #6625, .T. ) ;
#10240=CARTESIAN_POINT ( 'NONE',  ( -16.29350689640809691, 65.65569765742554864, 0.000000000000000000 ) ) ;
#10271=DIRECTION ( 'NONE',  ( -0.000000000000000000, -1.000000000000000000, -0.000000000000000000 ) ) ;
#10293=SHAPE_REPRESENTATION_RELATIONSHIP ( 'NONE' , 'NONE' ,  #3996, #2018 ) ;
#10295=DIRECTION ( 'NONE',  ( 0.000000000000000000, 0.000000000000000000, -1.000000000000000000 ) ) ;
#10296=FACE_OUTER_BOUND ( 'NONE', #8971, .T. ) ;
#10382=AXIS2_PLACEMENT_3D ( 'NONE', #2875, #2078, #5308 ) ;
#10383=PLANE ( 'NONE',  #4418 ) ;
#10397=ADVANCED_FACE ( 'NONE', ( #5087 ), #8911, .T. ) ;
#10418=EDGE_CURVE ( 'NONE', #9202, #7171, #8477, .T. ) ;
#10430=CARTESIAN_POINT ( 'NONE',  ( -16.29350689640809691, 11.33971203780352255, 0.000000000000000000 ) ) ;
#10433=DIRECTION ( 'NONE',  ( 0.000000000000000000, -0.000000000000000000, 1.000000000000000000 ) ) ;
#10435=PRODUCT_DEFINITION_SHAPE ( 'NONE', 'NONE',  #1785 ) ;
#10512=COLOUR_RGB('Grey',0.48,0.52,0.57);
#10513=FILL_AREA_STYLE_COLOUR('',#10512);
#10514=FILL_AREA_STYLE('',(#10513));
#10515=SURFACE_STYLE_FILL_AREA(#10514);
#10516=SURFACE_SIDE_STYLE('',(#10515));
#10517=SURFACE_STYLE_USAGE(.BOTH.,#10516);
#10518=PRESENTATION_STYLE_ASSIGNMENT((#10517));
ENDSEC;
END-ISO-10303-21;
